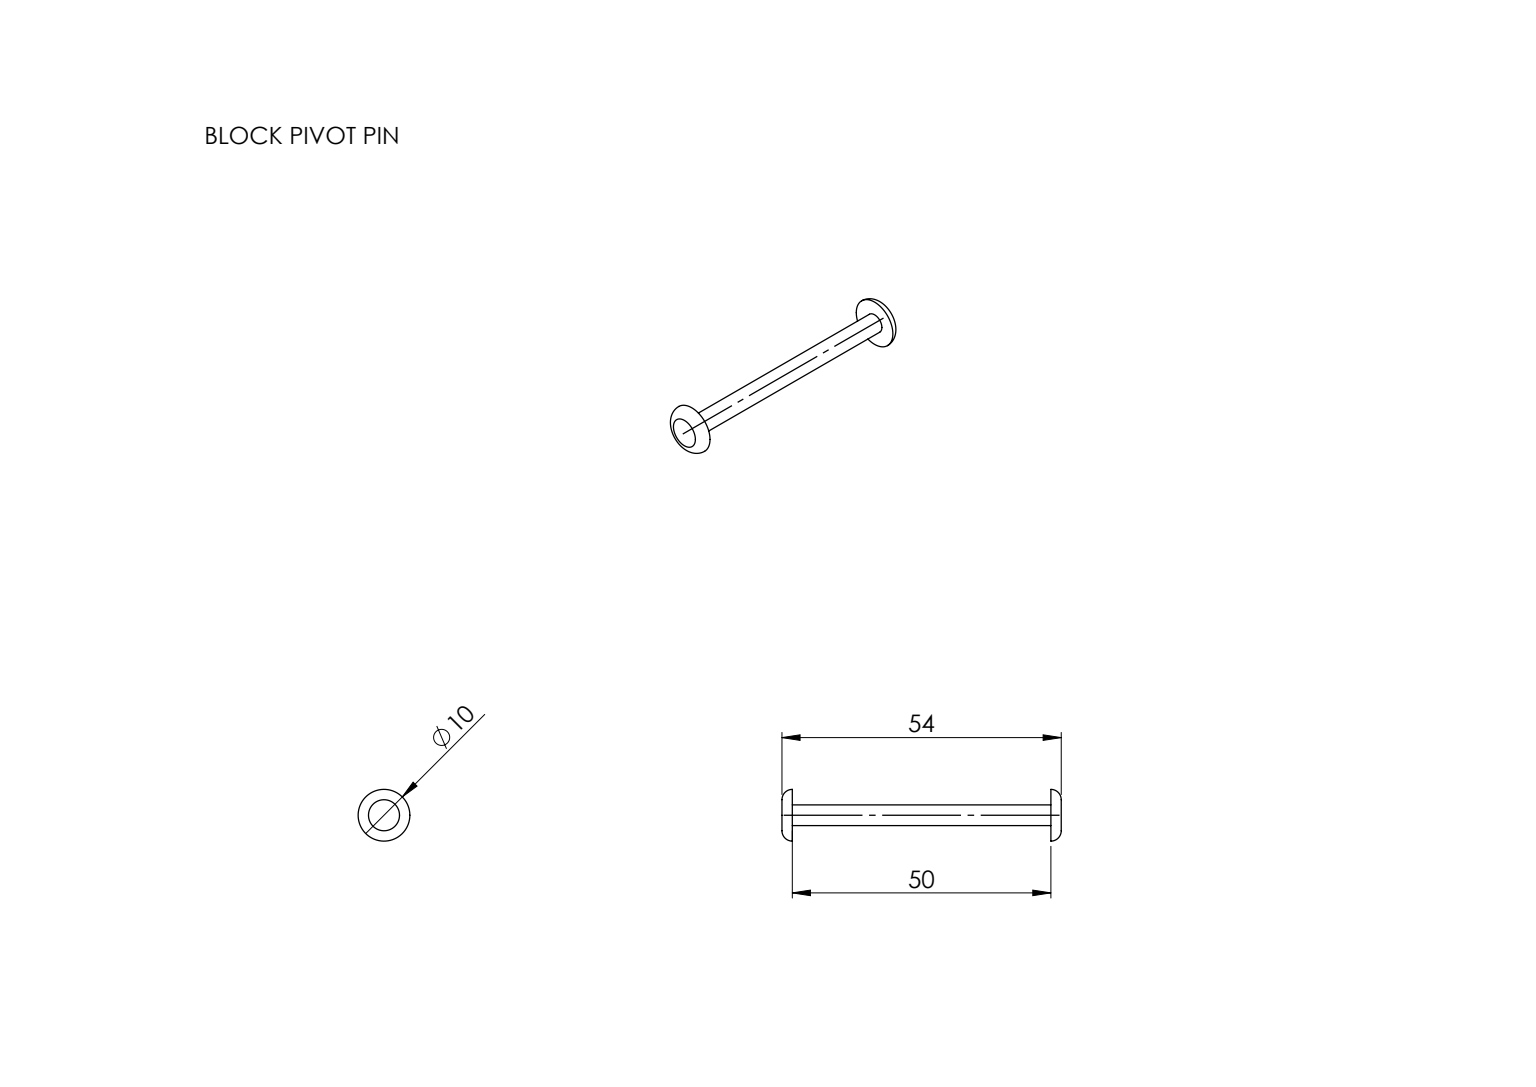
ISO-10303-21;
HEADER;
FILE_DESCRIPTION (('STEP AP214'),
    '1' );
FILE_NAME ('block pivot pin.step',
    '2026-10-02T13:02:33',
    ( '' ),
    ( '' ),
    'SwSTEP 2.0',
    'SolidWorks 2026',
    '' );
FILE_SCHEMA (( 'AUTOMOTIVE_DESIGN' ));
ENDSEC;

DATA;
#13=ORIENTED_EDGE ( 'NONE', *, *, #7836, .F. ) ;
#49=CARTESIAN_POINT ( 'NONE',  ( 0.000000000000000000, 0.000000000000000000, 32.00000000000000000 ) ) ;
#152=TOROIDAL_SURFACE ( 'NONE', #18040, 3.000000000000004441, 2.000000000000000000 ) ;
#162=FACE_OUTER_BOUND ( 'NONE', #5968, .T. ) ;
#199=EDGE_CURVE ( 'NONE', #827, #16818, #10252, .T. ) ;
#241=VERTEX_POINT ( 'NONE', #17685 ) ;
#284=CARTESIAN_POINT ( 'NONE',  ( 2.000000000000000000, 0.000000000000000000, 30.00000000000000000 ) ) ;
#347=AXIS2_PLACEMENT_3D ( 'NONE', #6635, #963, #6737 ) ;
#374=DIRECTION ( 'NONE',  ( 1.000000000000000000, 0.000000000000000000, 0.000000000000000000 ) ) ;
#421=PLANE ( 'NONE',  #6625 ) ;
#438=DIRECTION ( 'NONE',  ( 1.000000000000000000, 0.000000000000000000, 0.000000000000000000 ) ) ;
#440=ORIENTED_EDGE ( 'NONE', *, *, #10556, .F. ) ;
#457=FACE_OUTER_BOUND ( 'NONE', #12580, .T. ) ;
#534=( GEOMETRIC_REPRESENTATION_CONTEXT ( 3 ) GLOBAL_UNCERTAINTY_ASSIGNED_CONTEXT ( ( #9804 ) ) GLOBAL_UNIT_ASSIGNED_CONTEXT ( ( #13864, #16748, #10928 ) ) REPRESENTATION_CONTEXT ( 'NONE', 'WORKASPACE' ) );
#811=SHAPE_DEFINITION_REPRESENTATION ( #14086, #15677 ) ;
#827=VERTEX_POINT ( 'NONE', #5596 ) ;
#963=DIRECTION ( 'NONE',  ( 0.000000000000000000, 0.000000000000000000, 1.000000000000000000 ) ) ;
#977=CIRCLE ( 'NONE', #11525, 3.000000000000004441 ) ;
#1015=ADVANCED_FACE ( 'NONE', ( #2544 ), #14301, .T. ) ;
#1104=PRESENTATION_STYLE_ASSIGNMENT (( #9432 ) ) ;
#1122=ORIENTED_EDGE ( 'NONE', *, *, #6807, .F. ) ;
#1197=VECTOR ( 'NONE', #3987, 1000.000000000000000 ) ;
#1241=EDGE_LOOP ( 'NONE', ( #7462, #12015, #9169, #11444 ) ) ;
#1276=CIRCLE ( 'NONE', #7029, 2.000000000000000000 ) ;
#1366=ORIENTED_EDGE ( 'NONE', *, *, #4171, .T. ) ;
#1397=ADVANCED_FACE ( 'NONE', ( #13031 ), #4562, .T. ) ;
#1445=ADVANCED_BREP_SHAPE_REPRESENTATION ( '', ( #8651, #18772 ), #13228 ) ;
#1473=DIRECTION ( 'NONE',  ( 1.000000000000000000, 0.000000000000000000, 0.000000000000000000 ) ) ;
#1493=AXIS2_PLACEMENT_3D ( 'NONE', #14628, #11848, #16229 ) ;
#1542=UNCERTAINTY_MEASURE_WITH_UNIT (LENGTH_MEASURE( 1.000000000000000082E-05 ), #7891, 'distance_accuracy_value', 'NONE');
#1642=ORIENTED_EDGE ( 'NONE', *, *, #1797, .T. ) ;
#1783=CARTESIAN_POINT ( 'NONE',  ( 0.000000000000000000, 0.000000000000000000, 30.00000000000000000 ) ) ;
#1797=EDGE_CURVE ( 'NONE', #8732, #9690, #4574, .T. ) ;
#1894=DIRECTION ( 'NONE',  ( -1.000000000000000000, -1.224646799147353207E-16, 0.000000000000000000 ) ) ;
#2114=DIRECTION ( 'NONE',  ( -1.000000000000000000, 0.000000000000000000, 0.000000000000000000 ) ) ;
#2135=DIRECTION ( 'NONE',  ( -1.000000000000000000, 0.000000000000000000, -0.000000000000000000 ) ) ;
#2171=CARTESIAN_POINT ( 'NONE',  ( 0.000000000000000000, 0.000000000000000000, -20.00000000000000355 ) ) ;
#2228=PLANE ( 'NONE',  #7808 ) ;
#2324=AXIS2_PLACEMENT_3D ( 'NONE', #15019, #4685, #438 ) ;
#2381=CARTESIAN_POINT ( 'NONE',  ( 3.000000000000004441, 4.898587196589418745E-16, -22.00000000000000711 ) ) ;
#2448=ORIENTED_EDGE ( 'NONE', *, *, #16132, .T. ) ;
#2515=ORIENTED_EDGE ( 'NONE', *, *, #12515, .T. ) ;
#2544=FACE_OUTER_BOUND ( 'NONE', #15336, .T. ) ;
#2546=DIRECTION ( 'NONE',  ( 0.000000000000000000, 0.000000000000000000, -1.000000000000000000 ) ) ;
#2586=ADVANCED_FACE ( 'NONE', ( #7778 ), #10054, .T. ) ;
#2650=MECHANICAL_DESIGN_GEOMETRIC_PRESENTATION_REPRESENTATION('',(#3830),#534);
#2723=DIRECTION ( 'NONE',  ( 1.000000000000000000, 0.000000000000000000, 0.000000000000000000 ) ) ;
#2935=ORIENTED_EDGE ( 'NONE', *, *, #3430, .F. ) ;
#2943=AXIS2_PLACEMENT_3D ( 'NONE', #13566, #10718, #2114 ) ;
#3077=CIRCLE ( 'NONE', #5199, 2.000000000000000000 ) ;
#3107=DIRECTION ( 'NONE',  ( 0.000000000000000000, 0.000000000000000000, -1.000000000000000000 ) ) ;
#3212=CARTESIAN_POINT ( 'NONE',  ( 0.000000000000000000, 0.000000000000000000, -20.00000000000000355 ) ) ;
#3225=( NAMED_UNIT ( * ) SI_UNIT ( $, .STERADIAN. ) SOLID_ANGLE_UNIT ( ) );
#3244=APPLICATION_CONTEXT ( 'automotive_design' ) ;
#3269=EDGE_CURVE ( 'NONE', #5005, #13430, #10487, .T. ) ;
#3294=DIRECTION ( 'NONE',  ( -1.224646799147353207E-16, 1.000000000000000000, 0.000000000000000000 ) ) ;
#3376=CARTESIAN_POINT ( 'NONE',  ( 2.000000000000000000, 0.000000000000000000, -20.00000000000000355 ) ) ;
#3430=EDGE_CURVE ( 'NONE', #16818, #6018, #8993, .T. ) ;
#3671=CIRCLE ( 'NONE', #6127, 5.000000000000004441 ) ;
#3686=( GEOMETRIC_REPRESENTATION_CONTEXT ( 3 ) GLOBAL_UNCERTAINTY_ASSIGNED_CONTEXT ( ( #1542 ) ) GLOBAL_UNIT_ASSIGNED_CONTEXT ( ( #7891, #10795, #3225 ) ) REPRESENTATION_CONTEXT ( 'NONE', 'WORKASPACE' ) );
#3751=CARTESIAN_POINT ( 'NONE',  ( 0.000000000000000000, 0.000000000000000000, 32.00000000000000000 ) ) ;
#3830=STYLED_ITEM ( 'NONE', ( #1104 ), #1445 ) ;
#3987=DIRECTION ( 'NONE',  ( 0.000000000000000000, 0.000000000000000000, 1.000000000000000000 ) ) ;
#4001=STYLED_ITEM ( 'NONE', ( #9125 ), #8651 ) ;
#4132=CIRCLE ( 'NONE', #18098, 2.000000000000000000 ) ;
#4138=CARTESIAN_POINT ( 'NONE',  ( -3.000000000000000000, 3.673940397442059868E-16, 30.00000000000000000 ) ) ;
#4171=EDGE_CURVE ( 'NONE', #9690, #241, #12716, .T. ) ;
#4238=AXIS2_PLACEMENT_3D ( 'NONE', #3751, #16880, #8330 ) ;
#4339=DIRECTION ( 'NONE',  ( 1.224646799147353207E-16, 1.000000000000000000, -0.000000000000000000 ) ) ;
#4362=VERTEX_POINT ( 'NONE', #13634 ) ;
#4416=DIRECTION ( 'NONE',  ( 1.000000000000000000, 0.000000000000000000, 0.000000000000000000 ) ) ;
#4422=CARTESIAN_POINT ( 'NONE',  ( 5.000000000000004441, 6.123233995736772199E-16, -20.00000000000000355 ) ) ;
#4498=VECTOR ( 'NONE', #10905, 1000.000000000000000 ) ;
#4562=TOROIDAL_SURFACE ( 'NONE', #5482, 3.000000000000004441, 2.000000000000000000 ) ;
#4574=CIRCLE ( 'NONE', #5806, 2.000000000000001776 ) ;
#4685=DIRECTION ( 'NONE',  ( -1.547359998875406858E-16, 4.084688078942370972E-17, -1.000000000000000000 ) ) ;
#4727=UNCERTAINTY_MEASURE_WITH_UNIT (LENGTH_MEASURE( 1.000000000000000082E-05 ), #6132, 'distance_accuracy_value', 'NONE');
#4852=CIRCLE ( 'NONE', #7898, 5.000000000000000000 ) ;
#4889=AXIS2_PLACEMENT_3D ( 'NONE', #16205, #3294, #1894 ) ;
#4914=CARTESIAN_POINT ( 'NONE',  ( 0.000000000000000000, 0.000000000000000000, 30.00000000000000000 ) ) ;
#4920=DIRECTION ( 'NONE',  ( 1.000000000000000000, 0.000000000000000000, 0.000000000000000000 ) ) ;
#4966=CIRCLE ( 'NONE', #7423, 2.000000000000000000 ) ;
#5005=VERTEX_POINT ( 'NONE', #3376 ) ;
#5018=SURFACE_SIDE_STYLE ('',( #10633 ) ) ;
#5058=ORIENTED_EDGE ( 'NONE', *, *, #7707, .T. ) ;
#5103=DIRECTION ( 'NONE',  ( 1.000000000000000000, 0.000000000000000000, 0.000000000000000000 ) ) ;
#5166=SURFACE_SIDE_STYLE ('',( #12339 ) ) ;
#5199=AXIS2_PLACEMENT_3D ( 'NONE', #4914, #12000, #5103 ) ;
#5251=CARTESIAN_POINT ( 'NONE',  ( 3.000000000000000000, 0.000000000000000000, 32.00000000000000000 ) ) ;
#5306=PLANE ( 'NONE',  #7037 ) ;
#5423=EDGE_LOOP ( 'NONE', ( #440, #13 ) ) ;
#5429=ADVANCED_FACE ( 'NONE', ( #10398, #12159 ), #2228, .F. ) ;
#5431=CARTESIAN_POINT ( 'NONE',  ( 0.000000000000000000, 0.000000000000000000, 30.00000000000000000 ) ) ;
#5440=EDGE_LOOP ( 'NONE', ( #18127, #8867, #15413, #16755 ) ) ;
#5482=AXIS2_PLACEMENT_3D ( 'NONE', #16959, #15513, #9823 ) ;
#5518=DIRECTION ( 'NONE',  ( 1.000000000000000000, 0.000000000000000000, 0.000000000000000000 ) ) ;
#5596=CARTESIAN_POINT ( 'NONE',  ( -5.000000000000004441, 0.000000000000000000, -20.00000000000000355 ) ) ;
#5684=DIRECTION ( 'NONE',  ( 0.000000000000000000, 0.000000000000000000, -1.000000000000000000 ) ) ;
#5693=ADVANCED_FACE ( 'NONE', ( #14812, #6402 ), #421, .F. ) ;
#5725=EDGE_CURVE ( 'NONE', #5005, #8991, #6677, .T. ) ;
#5777=CARTESIAN_POINT ( 'NONE',  ( 0.000000000000000000, 0.000000000000000000, 30.00000000000000000 ) ) ;
#5806=AXIS2_PLACEMENT_3D ( 'NONE', #18527, #10114, #5684 ) ;
#5968=EDGE_LOOP ( 'NONE', ( #6770, #17857, #12043, #15501 ) ) ;
#6015=ORIENTED_EDGE ( 'NONE', *, *, #10077, .T. ) ;
#6018=VERTEX_POINT ( 'NONE', #2381 ) ;
#6127=AXIS2_PLACEMENT_3D ( 'NONE', #15225, #8222, #17056 ) ;
#6132=( LENGTH_UNIT ( ) NAMED_UNIT ( * ) SI_UNIT ( .MILLI., .METRE. ) );
#6206=CARTESIAN_POINT ( 'NONE',  ( 0.000000000000000000, 0.000000000000000000, 30.00000000000000000 ) ) ;
#6378=CARTESIAN_POINT ( 'NONE',  ( 0.000000000000000000, 0.000000000000000000, 30.00000000000000000 ) ) ;
#6393=FILL_AREA_STYLE_COLOUR ( '', #13089 ) ;
#6402=FACE_OUTER_BOUND ( 'NONE', #13109, .T. ) ;
#6625=AXIS2_PLACEMENT_3D ( 'NONE', #6206, #11932, #17783 ) ;
#6635=CARTESIAN_POINT ( 'NONE',  ( 0.000000000000000000, 0.000000000000000000, -25.65685424949237614 ) ) ;
#6668=ORIENTED_EDGE ( 'NONE', *, *, #8015, .T. ) ;
#6677=LINE ( 'NONE', #18461, #4498 ) ;
#6737=DIRECTION ( 'NONE',  ( 1.000000000000000000, 0.000000000000000000, 0.000000000000000000 ) ) ;
#6770=ORIENTED_EDGE ( 'NONE', *, *, #16936, .F. ) ;
#6807=EDGE_CURVE ( 'NONE', #8991, #4362, #4132, .T. ) ;
#6866=ORIENTED_EDGE ( 'NONE', *, *, #10556, .T. ) ;
#6906=COLOUR_RGB ( '', 0.40784314, 0.44705882, 0.49803922) ;
#7029=AXIS2_PLACEMENT_3D ( 'NONE', #4138, #4339, #14481 ) ;
#7037=AXIS2_PLACEMENT_3D ( 'NONE', #15615, #9670, #12398 ) ;
#7175=DIRECTION ( 'NONE',  ( 1.000000000000000000, 0.000000000000000000, 0.000000000000000000 ) ) ;
#7292=CYLINDRICAL_SURFACE ( 'NONE', #14264, 2.000000000000000000 ) ;
#7423=AXIS2_PLACEMENT_3D ( 'NONE', #3212, #15253, #2723 ) ;
#7462=ORIENTED_EDGE ( 'NONE', *, *, #7707, .F. ) ;
#7473=DIRECTION ( 'NONE',  ( 0.000000000000000000, 0.000000000000000000, 1.000000000000000000 ) ) ;
#7560=ORIENTED_EDGE ( 'NONE', *, *, #16132, .F. ) ;
#7572=DIRECTION ( 'NONE',  ( 0.000000000000000000, 0.000000000000000000, 1.000000000000000000 ) ) ;
#7707=EDGE_CURVE ( 'NONE', #8225, #6018, #14876, .T. ) ;
#7769=PRODUCT_DEFINITION_CONTEXT ( 'detailed design', #3244, 'design' ) ;
#7778=FACE_OUTER_BOUND ( 'NONE', #5440, .T. ) ;
#7808=AXIS2_PLACEMENT_3D ( 'NONE', #10313, #3107, #2135 ) ;
#7836=EDGE_CURVE ( 'NONE', #8225, #827, #14300, .T. ) ;
#7876=DIRECTION ( 'NONE',  ( 0.000000000000000000, 0.000000000000000000, -1.000000000000000000 ) ) ;
#7891=( LENGTH_UNIT ( ) NAMED_UNIT ( * ) SI_UNIT ( .MILLI., .METRE. ) );
#7898=AXIS2_PLACEMENT_3D ( 'NONE', #5777, #8614, #14386 ) ;
#7974=ADVANCED_FACE ( 'NONE', ( #16688 ), #13803, .T. ) ;
#8001=PRODUCT_CONTEXT ( 'NONE', #16966, 'mechanical' ) ;
#8015=EDGE_CURVE ( 'NONE', #6018, #16818, #977, .T. ) ;
#8036=EDGE_CURVE ( 'NONE', #10693, #241, #1276, .T. ) ;
#8222=DIRECTION ( 'NONE',  ( 0.000000000000000000, 0.000000000000000000, -1.000000000000000000 ) ) ;
#8225=VERTEX_POINT ( 'NONE', #4422 ) ;
#8330=DIRECTION ( 'NONE',  ( 1.000000000000000000, 0.000000000000000000, -0.000000000000000000 ) ) ;
#8407=EDGE_LOOP ( 'NONE', ( #16320, #6668 ) ) ;
#8443=CLOSED_SHELL ( 'NONE', ( #2586, #1397, #7974, #16024, #1015, #5693, #10181, #5429, #13190, #14541 ) ) ;
#8519=ORIENTED_EDGE ( 'NONE', *, *, #16833, .F. ) ;
#8529=DIRECTION ( 'NONE',  ( -1.000000000000000000, 0.000000000000000000, 0.000000000000000000 ) ) ;
#8614=DIRECTION ( 'NONE',  ( 0.000000000000000000, 0.000000000000000000, 1.000000000000000000 ) ) ;
#8651=MANIFOLD_SOLID_BREP ( 'Fillet1', #8443 ) ;
#8732=VERTEX_POINT ( 'NONE', #12693 ) ;
#8738=LINE ( 'NONE', #13093, #1197 ) ;
#8757=ORIENTED_EDGE ( 'NONE', *, *, #8036, .F. ) ;
#8867=ORIENTED_EDGE ( 'NONE', *, *, #8036, .T. ) ;
#8873=CARTESIAN_POINT ( 'NONE',  ( -5.000000000000000000, 6.123233995736766282E-16, 30.00000000000000000 ) ) ;
#8991=VERTEX_POINT ( 'NONE', #284 ) ;
#8993=CIRCLE ( 'NONE', #2943, 3.000000000000004441 ) ;
#9087=AXIS2_PLACEMENT_3D ( 'NONE', #18594, #15507, #7175 ) ;
#9125=PRESENTATION_STYLE_ASSIGNMENT (( #14899 ) ) ;
#9169=ORIENTED_EDGE ( 'NONE', *, *, #199, .T. ) ;
#9336=CIRCLE ( 'NONE', #17853, 5.000000000000000000 ) ;
#9432=SURFACE_STYLE_USAGE ( .BOTH. , #5166 ) ;
#9507=DIRECTION ( 'NONE',  ( 0.000000000000000000, 0.000000000000000000, 1.000000000000000000 ) ) ;
#9670=DIRECTION ( 'NONE',  ( 0.000000000000000000, 0.000000000000000000, -1.000000000000000000 ) ) ;
#9690=VERTEX_POINT ( 'NONE', #5251 ) ;
#9704=EDGE_LOOP ( 'NONE', ( #14746, #13830 ) ) ;
#9716=AXIS2_PLACEMENT_3D ( 'NONE', #49, #14445, #1473 ) ;
#9804=UNCERTAINTY_MEASURE_WITH_UNIT (LENGTH_MEASURE( 1.000000000000000082E-05 ), #13864, 'distance_accuracy_value', 'NONE');
#9823=DIRECTION ( 'NONE',  ( -1.000000000000000000, 0.000000000000000000, 0.000000000000000000 ) ) ;
#9883=TOROIDAL_SURFACE ( 'NONE', #18411, 3.000000000000000000, 2.000000000000000000 ) ;
#9913=DIRECTION ( 'NONE',  ( -1.000000000000000000, 0.000000000000000000, 0.000000000000000000 ) ) ;
#10012=CARTESIAN_POINT ( 'NONE',  ( 0.000000000000000000, 0.000000000000000000, -20.00000000000000355 ) ) ;
#10054=TOROIDAL_SURFACE ( 'NONE', #13668, 3.000000000000000000, 2.000000000000000000 ) ;
#10077=EDGE_CURVE ( 'NONE', #4362, #8991, #3077, .T. ) ;
#10114=DIRECTION ( 'NONE',  ( 0.000000000000000000, -1.000000000000000000, 0.000000000000000000 ) ) ;
#10181=ADVANCED_FACE ( 'NONE', ( #15536 ), #5306, .T. ) ;
#10187=CARTESIAN_POINT ( 'NONE',  ( -2.000000000000000000, 2.449293598294706414E-16, -20.00000000000000355 ) ) ;
#10190=CARTESIAN_POINT ( 'NONE',  ( 0.000000000000000000, 0.000000000000000000, -25.65685424949237614 ) ) ;
#10252=CIRCLE ( 'NONE', #1493, 2.000000000000001776 ) ;
#10313=CARTESIAN_POINT ( 'NONE',  ( 0.000000000000000000, 0.000000000000000000, -20.00000000000000355 ) ) ;
#10398=FACE_BOUND ( 'NONE', #9704, .T. ) ;
#10487=CIRCLE ( 'NONE', #2324, 2.000000000000000000 ) ;
#10556=EDGE_CURVE ( 'NONE', #827, #8225, #3671, .T. ) ;
#10633=SURFACE_STYLE_FILL_AREA ( #16232 ) ;
#10658=FILL_AREA_STYLE_COLOUR ( '', #6906 ) ;
#10693=VERTEX_POINT ( 'NONE', #8873 ) ;
#10718=DIRECTION ( 'NONE',  ( 0.000000000000000000, 0.000000000000000000, -1.000000000000000000 ) ) ;
#10795=( NAMED_UNIT ( * ) PLANE_ANGLE_UNIT ( ) SI_UNIT ( $, .RADIAN. ) );
#10905=DIRECTION ( 'NONE',  ( 0.000000000000000000, 0.000000000000000000, 1.000000000000000000 ) ) ;
#10928=( NAMED_UNIT ( * ) SI_UNIT ( $, .STERADIAN. ) SOLID_ANGLE_UNIT ( ) );
#11075=ORIENTED_EDGE ( 'NONE', *, *, #13168, .F. ) ;
#11155=DIRECTION ( 'NONE',  ( -1.000000000000000000, 0.000000000000000000, 0.000000000000000000 ) ) ;
#11363=PRODUCT_DEFINITION ( 'UNKNOWN', '', #15965, #7769 ) ;
#11444=ORIENTED_EDGE ( 'NONE', *, *, #8015, .F. ) ;
#11489=CIRCLE ( 'NONE', #9716, 3.000000000000000000 ) ;
#11525=AXIS2_PLACEMENT_3D ( 'NONE', #17439, #2546, #8529 ) ;
#11718=EDGE_LOOP ( 'NONE', ( #6866, #5058, #2935, #17155 ) ) ;
#11848=DIRECTION ( 'NONE',  ( -0.000000000000000000, -1.000000000000000000, -0.000000000000000000 ) ) ;
#11918=ORIENTED_EDGE ( 'NONE', *, *, #16936, .T. ) ;
#11932=DIRECTION ( 'NONE',  ( 0.000000000000000000, 0.000000000000000000, 1.000000000000000000 ) ) ;
#11951=( NAMED_UNIT ( * ) PLANE_ANGLE_UNIT ( ) SI_UNIT ( $, .RADIAN. ) );
#11962=ORIENTED_EDGE ( 'NONE', *, *, #6807, .T. ) ;
#12000=DIRECTION ( 'NONE',  ( 0.000000000000000000, 0.000000000000000000, 1.000000000000000000 ) ) ;
#12015=ORIENTED_EDGE ( 'NONE', *, *, #7836, .T. ) ;
#12043=ORIENTED_EDGE ( 'NONE', *, *, #5725, .T. ) ;
#12159=FACE_OUTER_BOUND ( 'NONE', #5423, .T. ) ;
#12237=ORIENTED_EDGE ( 'NONE', *, *, #5725, .F. ) ;
#12285=DIRECTION ( 'NONE',  ( 0.000000000000000000, 0.000000000000000000, -1.000000000000000000 ) ) ;
#12339=SURFACE_STYLE_FILL_AREA ( #18189 ) ;
#12398=DIRECTION ( 'NONE',  ( -1.000000000000000000, 0.000000000000000000, -0.000000000000000000 ) ) ;
#12452=SHAPE_REPRESENTATION_RELATIONSHIP ( 'NONE' , 'NONE' ,  #15677, #1445 ) ;
#12515=EDGE_CURVE ( 'NONE', #241, #9690, #11489, .T. ) ;
#12580=EDGE_LOOP ( 'NONE', ( #8757, #2448, #1642, #16975 ) ) ;
#12689=CARTESIAN_POINT ( 'NONE',  ( 0.000000000000000000, 0.000000000000000000, 30.00000000000000000 ) ) ;
#12693=CARTESIAN_POINT ( 'NONE',  ( 5.000000000000000000, 0.000000000000000000, 30.00000000000000000 ) ) ;
#12716=CIRCLE ( 'NONE', #9087, 3.000000000000000000 ) ;
#12720=EDGE_LOOP ( 'NONE', ( #11075, #11918, #1122, #12237 ) ) ;
#13031=FACE_OUTER_BOUND ( 'NONE', #11718, .T. ) ;
#13089=COLOUR_RGB ( '', 0.40784314, 0.44705882, 0.49803922) ;
#13093=CARTESIAN_POINT ( 'NONE',  ( -2.000000000000000000, 2.449293598294706414E-16, -25.65685424949237614 ) ) ;
#13109=EDGE_LOOP ( 'NONE', ( #8519, #7560 ) ) ;
#13168=EDGE_CURVE ( 'NONE', #13430, #5005, #4966, .T. ) ;
#13190=ADVANCED_FACE ( 'NONE', ( #15810 ), #152, .T. ) ;
#13228=( GEOMETRIC_REPRESENTATION_CONTEXT ( 3 ) GLOBAL_UNCERTAINTY_ASSIGNED_CONTEXT ( ( #4727 ) ) GLOBAL_UNIT_ASSIGNED_CONTEXT ( ( #6132, #11951, #16255 ) ) REPRESENTATION_CONTEXT ( 'NONE', 'WORKASPACE' ) );
#13381=MECHANICAL_DESIGN_GEOMETRIC_PRESENTATION_REPRESENTATION('',(#4001),#3686);
#13430=VERTEX_POINT ( 'NONE', #10187 ) ;
#13566=CARTESIAN_POINT ( 'NONE',  ( 0.000000000000000000, 0.000000000000000000, -22.00000000000000711 ) ) ;
#13611=CARTESIAN_POINT ( 'NONE',  ( 0.000000000000000000, 0.000000000000000000, 0.000000000000000000 ) ) ;
#13634=CARTESIAN_POINT ( 'NONE',  ( -2.000000000000000000, 2.449293598294706414E-16, 30.00000000000000000 ) ) ;
#13668=AXIS2_PLACEMENT_3D ( 'NONE', #6378, #17955, #4920 ) ;
#13803=CYLINDRICAL_SURFACE ( 'NONE', #347, 2.000000000000000000 ) ;
#13830=ORIENTED_EDGE ( 'NONE', *, *, #13168, .T. ) ;
#13864=( LENGTH_UNIT ( ) NAMED_UNIT ( * ) SI_UNIT ( .MILLI., .METRE. ) );
#14086=PRODUCT_DEFINITION_SHAPE ( 'NONE', 'NONE',  #11363 ) ;
#14264=AXIS2_PLACEMENT_3D ( 'NONE', #10190, #17149, #4416 ) ;
#14300=CIRCLE ( 'NONE', #17652, 5.000000000000004441 ) ;
#14301=PLANE ( 'NONE',  #4238 ) ;
#14386=DIRECTION ( 'NONE',  ( 1.000000000000000000, 0.000000000000000000, 0.000000000000000000 ) ) ;
#14445=DIRECTION ( 'NONE',  ( 0.000000000000000000, 0.000000000000000000, 1.000000000000000000 ) ) ;
#14481=DIRECTION ( 'NONE',  ( -1.000000000000000000, 1.224646799147353207E-16, 0.000000000000000000 ) ) ;
#14541=ADVANCED_FACE ( 'NONE', ( #457 ), #9883, .T. ) ;
#14628=CARTESIAN_POINT ( 'NONE',  ( -3.000000000000004441, 0.000000000000000000, -20.00000000000000355 ) ) ;
#14746=ORIENTED_EDGE ( 'NONE', *, *, #3269, .T. ) ;
#14759=DIRECTION ( 'NONE',  ( 1.000000000000000000, 0.000000000000000000, 0.000000000000000000 ) ) ;
#14812=FACE_BOUND ( 'NONE', #17333, .T. ) ;
#14876=CIRCLE ( 'NONE', #4889, 2.000000000000000000 ) ;
#14899=SURFACE_STYLE_USAGE ( .BOTH. , #5018 ) ;
#15019=CARTESIAN_POINT ( 'NONE',  ( 0.000000000000000000, 0.000000000000000000, -20.00000000000000355 ) ) ;
#15225=CARTESIAN_POINT ( 'NONE',  ( 0.000000000000000000, 0.000000000000000000, -20.00000000000000355 ) ) ;
#15253=DIRECTION ( 'NONE',  ( -1.547359998875406858E-16, 4.084688078942370972E-17, -1.000000000000000000 ) ) ;
#15287=PRODUCT ( 'block pivot pin', 'block pivot pin', '', ( #8001 ) ) ;
#15336=EDGE_LOOP ( 'NONE', ( #1366, #2515 ) ) ;
#15413=ORIENTED_EDGE ( 'NONE', *, *, #4171, .F. ) ;
#15477=DIRECTION ( 'NONE',  ( 1.000000000000000000, 0.000000000000000000, 0.000000000000000000 ) ) ;
#15501=ORIENTED_EDGE ( 'NONE', *, *, #10077, .F. ) ;
#15507=DIRECTION ( 'NONE',  ( 0.000000000000000000, 0.000000000000000000, 1.000000000000000000 ) ) ;
#15513=DIRECTION ( 'NONE',  ( 0.000000000000000000, 0.000000000000000000, -1.000000000000000000 ) ) ;
#15536=FACE_OUTER_BOUND ( 'NONE', #8407, .T. ) ;
#15615=CARTESIAN_POINT ( 'NONE',  ( 0.000000000000000000, 0.000000000000000000, -22.00000000000000711 ) ) ;
#15677=SHAPE_REPRESENTATION ( 'block pivot pin', ( #18772 ), #13228 ) ;
#15810=FACE_OUTER_BOUND ( 'NONE', #1241, .T. ) ;
#15965=PRODUCT_DEFINITION_FORMATION_WITH_SPECIFIED_SOURCE ( 'ANY', '', #15287, .NOT_KNOWN. ) ;
#16024=ADVANCED_FACE ( 'NONE', ( #162 ), #7292, .T. ) ;
#16132=EDGE_CURVE ( 'NONE', #10693, #8732, #4852, .T. ) ;
#16205=CARTESIAN_POINT ( 'NONE',  ( 3.000000000000004441, 3.673940397442064798E-16, -20.00000000000000355 ) ) ;
#16229=DIRECTION ( 'NONE',  ( 0.000000000000000000, 0.000000000000000000, -1.000000000000000000 ) ) ;
#16232=FILL_AREA_STYLE ('',( #6393 ) ) ;
#16255=( NAMED_UNIT ( * ) SI_UNIT ( $, .STERADIAN. ) SOLID_ANGLE_UNIT ( ) );
#16320=ORIENTED_EDGE ( 'NONE', *, *, #3430, .T. ) ;
#16688=FACE_OUTER_BOUND ( 'NONE', #12720, .T. ) ;
#16748=( NAMED_UNIT ( * ) PLANE_ANGLE_UNIT ( ) SI_UNIT ( $, .RADIAN. ) );
#16755=ORIENTED_EDGE ( 'NONE', *, *, #1797, .F. ) ;
#16818=VERTEX_POINT ( 'NONE', #18465 ) ;
#16833=EDGE_CURVE ( 'NONE', #8732, #10693, #9336, .T. ) ;
#16880=DIRECTION ( 'NONE',  ( 0.000000000000000000, 0.000000000000000000, 1.000000000000000000 ) ) ;
#16936=EDGE_CURVE ( 'NONE', #13430, #4362, #8738, .T. ) ;
#16959=CARTESIAN_POINT ( 'NONE',  ( 0.000000000000000000, 0.000000000000000000, -20.00000000000000355 ) ) ;
#16966=APPLICATION_CONTEXT ( 'automotive_design' ) ;
#16975=ORIENTED_EDGE ( 'NONE', *, *, #12515, .F. ) ;
#17056=DIRECTION ( 'NONE',  ( -1.000000000000000000, 0.000000000000000000, 0.000000000000000000 ) ) ;
#17149=DIRECTION ( 'NONE',  ( 0.000000000000000000, 0.000000000000000000, 1.000000000000000000 ) ) ;
#17155=ORIENTED_EDGE ( 'NONE', *, *, #199, .F. ) ;
#17333=EDGE_LOOP ( 'NONE', ( #11962, #6015 ) ) ;
#17439=CARTESIAN_POINT ( 'NONE',  ( 0.000000000000000000, 0.000000000000000000, -22.00000000000000711 ) ) ;
#17652=AXIS2_PLACEMENT_3D ( 'NONE', #2171, #12285, #11155 ) ;
#17685=CARTESIAN_POINT ( 'NONE',  ( -3.000000000000000000, 4.898587196589412829E-16, 32.00000000000000000 ) ) ;
#17783=DIRECTION ( 'NONE',  ( 1.000000000000000000, 0.000000000000000000, -0.000000000000000000 ) ) ;
#17853=AXIS2_PLACEMENT_3D ( 'NONE', #5431, #9507, #15477 ) ;
#17857=ORIENTED_EDGE ( 'NONE', *, *, #3269, .F. ) ;
#17955=DIRECTION ( 'NONE',  ( 0.000000000000000000, 0.000000000000000000, 1.000000000000000000 ) ) ;
#18040=AXIS2_PLACEMENT_3D ( 'NONE', #10012, #7876, #9913 ) ;
#18098=AXIS2_PLACEMENT_3D ( 'NONE', #12689, #18547, #5518 ) ;
#18127=ORIENTED_EDGE ( 'NONE', *, *, #16833, .T. ) ;
#18189=FILL_AREA_STYLE ('',( #10658 ) ) ;
#18411=AXIS2_PLACEMENT_3D ( 'NONE', #1783, #7572, #374 ) ;
#18461=CARTESIAN_POINT ( 'NONE',  ( 2.000000000000000000, 0.000000000000000000, -25.65685424949237614 ) ) ;
#18465=CARTESIAN_POINT ( 'NONE',  ( -3.000000000000004441, 0.000000000000000000, -22.00000000000000711 ) ) ;
#18527=CARTESIAN_POINT ( 'NONE',  ( 3.000000000000000000, 0.000000000000000000, 30.00000000000000000 ) ) ;
#18547=DIRECTION ( 'NONE',  ( 0.000000000000000000, 0.000000000000000000, 1.000000000000000000 ) ) ;
#18594=CARTESIAN_POINT ( 'NONE',  ( 0.000000000000000000, 0.000000000000000000, 32.00000000000000000 ) ) ;
#18772=AXIS2_PLACEMENT_3D ( 'NONE', #13611, #7473, #14759 ) ;
ENDSEC;
END-ISO-10303-21;
